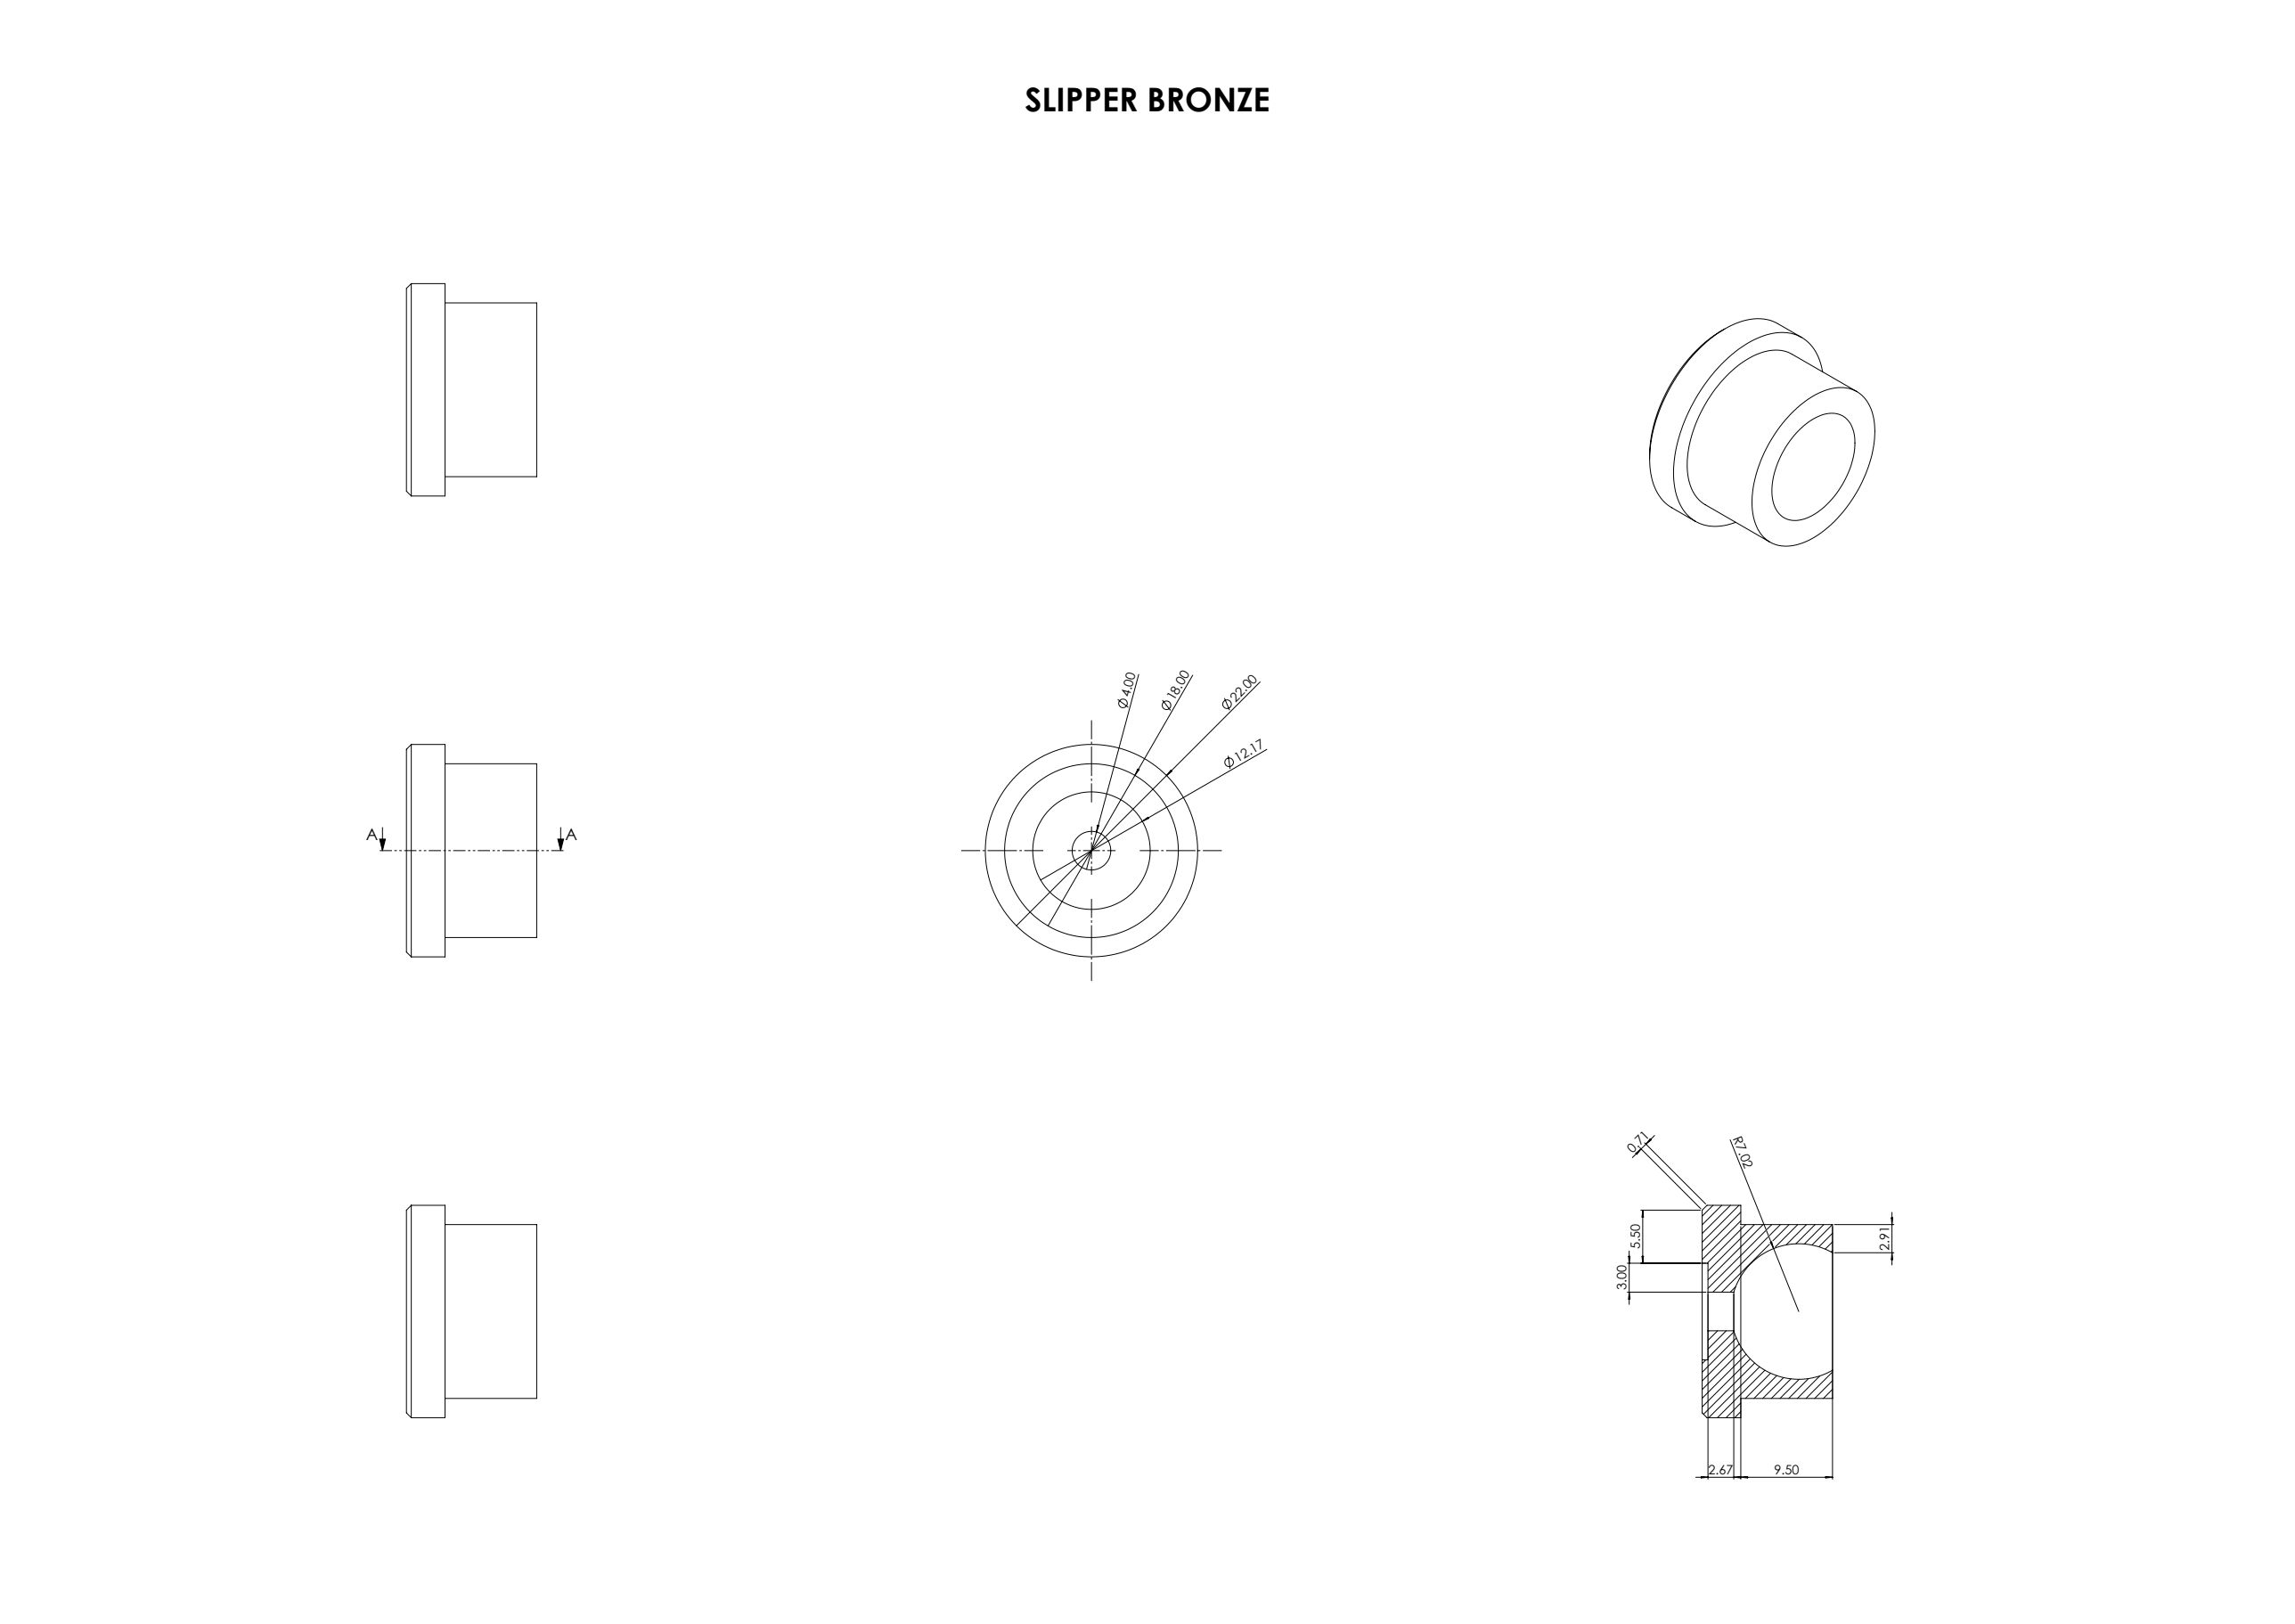
ISO-10303-21;
HEADER;
/* Generated by software containing ST-Developer
 * from STEP Tools, Inc. (www.steptools.com) 
 */

FILE_DESCRIPTION(
/* description */ (''),
/* implementation_level */ '2;1');

FILE_NAME(
/* name */ '06_Slipper_Bronze.step',
/* time_stamp */ '2026-10-26T07:49:00-07:00',
/* author */ (''),
/* organization */ (''),
/* preprocessor_version */ 'ST-DEVELOPER v20.2',
/* originating_system */ 'Autodesk Translation Framework v15.15.0.0',
/* authorisation */ '');

FILE_SCHEMA (('AUTOMOTIVE_DESIGN { 1 0 10303 214 3 1 1 }'));
ENDSEC;

DATA;
#10=MECHANICAL_DESIGN_GEOMETRIC_PRESENTATION_REPRESENTATION('',(#188),#38507);
#146=SPHERICAL_SURFACE('',#16295,7.02);
#158=SHAPE_REPRESENTATION_RELATIONSHIP('SRR','None',#38586,#173);
#173=ADVANCED_BREP_SHAPE_REPRESENTATION('',(#203),#38503);
#188=STYLED_ITEM('',(#38713),#203);
#203=MANIFOLD_SOLID_BREP('Slipper_Body',#15082);
#510=FACE_BOUND('',#3163,.T.);
#511=FACE_BOUND('',#3167,.T.);
#512=FACE_BOUND('',#3170,.T.);
#513=FACE_BOUND('',#3172,.T.);
#514=FACE_BOUND('',#3175,.T.);
#805=PLANE('',#16283);
#806=PLANE('',#16289);
#807=PLANE('',#16293);
#808=PLANE('',#16303);
#1509=CYLINDRICAL_SURFACE('',#16280,5.);
#1510=CYLINDRICAL_SURFACE('',#16287,11.);
#1511=CYLINDRICAL_SURFACE('',#16291,9.);
#1512=CYLINDRICAL_SURFACE('',#16301,2.);
#2181=FACE_OUTER_BOUND('',#3161,.T.);
#2182=FACE_OUTER_BOUND('',#3162,.T.);
#2183=FACE_OUTER_BOUND('',#3164,.T.);
#2184=FACE_OUTER_BOUND('',#3165,.T.);
#2185=FACE_OUTER_BOUND('',#3166,.T.);
#2186=FACE_OUTER_BOUND('',#3168,.T.);
#2187=FACE_OUTER_BOUND('',#3169,.T.);
#2188=FACE_OUTER_BOUND('',#3171,.T.);
#2189=FACE_OUTER_BOUND('',#3173,.T.);
#2190=FACE_OUTER_BOUND('',#3174,.T.);
#3161=EDGE_LOOP('',(#12527,#12528,#12529,#12530));
#3162=EDGE_LOOP('',(#12531));
#3163=EDGE_LOOP('',(#12532));
#3164=EDGE_LOOP('',(#12533,#12534,#12535,#12536));
#3165=EDGE_LOOP('',(#12537,#12538,#12539,#12540));
#3166=EDGE_LOOP('',(#12541));
#3167=EDGE_LOOP('',(#12542));
#3168=EDGE_LOOP('',(#12543,#12544,#12545,#12546));
#3169=EDGE_LOOP('',(#12547));
#3170=EDGE_LOOP('',(#12548));
#3171=EDGE_LOOP('',(#12549,#12550,#12551,#12552,#12553,#12554,#12555));
#3172=EDGE_LOOP('',(#12556));
#3173=EDGE_LOOP('',(#12557,#12558,#12559,#12560,#12561,#12562));
#3174=EDGE_LOOP('',(#12563));
#3175=EDGE_LOOP('',(#12564));
#4136=LINE('',#27087,#5205);
#4137=LINE('',#27095,#5206);
#4138=LINE('',#27099,#5207);
#4139=LINE('',#27106,#5208);
#4140=LINE('',#27123,#5209);
#5205=VECTOR('',#19439,5.);
#5206=VECTOR('',#19450,10.75);
#5207=VECTOR('',#19455,11.);
#5208=VECTOR('',#19464,9.);
#5209=VECTOR('',#19483,2.);
#6128=CIRCLE('',#16281,5.);
#6129=CIRCLE('',#16282,5.);
#6130=CIRCLE('',#16284,10.5);
#6131=CIRCLE('',#16286,11.);
#6132=CIRCLE('',#16288,11.);
#6133=CIRCLE('',#16290,9.);
#6134=CIRCLE('',#16292,9.);
#6135=CIRCLE('',#16294,6.08526088183572);
#6136=CIRCLE('',#16296,2.);
#6137=CIRCLE('',#16297,7.02);
#6138=CIRCLE('',#16298,2.);
#6139=CIRCLE('',#16299,2.);
#6140=CIRCLE('',#16300,7.02);
#6141=CIRCLE('',#16302,2.);
#7132=VERTEX_POINT('',#27084);
#7133=VERTEX_POINT('',#27086);
#7134=VERTEX_POINT('',#27090);
#7135=VERTEX_POINT('',#27093);
#7136=VERTEX_POINT('',#27097);
#7137=VERTEX_POINT('',#27101);
#7138=VERTEX_POINT('',#27104);
#7139=VERTEX_POINT('',#27108);
#7140=VERTEX_POINT('',#27111);
#7141=VERTEX_POINT('',#27112);
#7142=VERTEX_POINT('',#27114);
#7143=VERTEX_POINT('',#27116);
#7144=VERTEX_POINT('',#27119);
#7145=VERTEX_POINT('',#27122);
#9012=EDGE_CURVE('',#7132,#7132,#6128,.T.);
#9013=EDGE_CURVE('',#7132,#7133,#4136,.T.);
#9014=EDGE_CURVE('',#7133,#7133,#6129,.T.);
#9015=EDGE_CURVE('',#7134,#7134,#6130,.T.);
#9016=EDGE_CURVE('',#7135,#7135,#6131,.T.);
#9017=EDGE_CURVE('',#7135,#7134,#4137,.T.);
#9018=EDGE_CURVE('',#7136,#7136,#6132,.T.);
#9019=EDGE_CURVE('',#7136,#7135,#4138,.T.);
#9020=EDGE_CURVE('',#7137,#7137,#6133,.T.);
#9021=EDGE_CURVE('',#7138,#7138,#6134,.T.);
#9022=EDGE_CURVE('',#7138,#7137,#4139,.T.);
#9023=EDGE_CURVE('',#7139,#7139,#6135,.T.);
#9024=EDGE_CURVE('',#7140,#7141,#6136,.T.);
#9025=EDGE_CURVE('',#7140,#7142,#6137,.T.);
#9026=EDGE_CURVE('',#7143,#7140,#6138,.T.);
#9027=EDGE_CURVE('',#7141,#7143,#6139,.T.);
#9028=EDGE_CURVE('',#7144,#7141,#6140,.T.);
#9029=EDGE_CURVE('',#7143,#7145,#4140,.T.);
#9030=EDGE_CURVE('',#7145,#7145,#6141,.T.);
#12527=ORIENTED_EDGE('',*,*,#9012,.T.);
#12528=ORIENTED_EDGE('',*,*,#9013,.T.);
#12529=ORIENTED_EDGE('',*,*,#9014,.F.);
#12530=ORIENTED_EDGE('',*,*,#9013,.F.);
#12531=ORIENTED_EDGE('',*,*,#9015,.F.);
#12532=ORIENTED_EDGE('',*,*,#9014,.T.);
#12533=ORIENTED_EDGE('',*,*,#9016,.F.);
#12534=ORIENTED_EDGE('',*,*,#9017,.T.);
#12535=ORIENTED_EDGE('',*,*,#9015,.T.);
#12536=ORIENTED_EDGE('',*,*,#9017,.F.);
#12537=ORIENTED_EDGE('',*,*,#9018,.F.);
#12538=ORIENTED_EDGE('',*,*,#9019,.T.);
#12539=ORIENTED_EDGE('',*,*,#9016,.T.);
#12540=ORIENTED_EDGE('',*,*,#9019,.F.);
#12541=ORIENTED_EDGE('',*,*,#9018,.T.);
#12542=ORIENTED_EDGE('',*,*,#9020,.F.);
#12543=ORIENTED_EDGE('',*,*,#9021,.F.);
#12544=ORIENTED_EDGE('',*,*,#9022,.T.);
#12545=ORIENTED_EDGE('',*,*,#9020,.T.);
#12546=ORIENTED_EDGE('',*,*,#9022,.F.);
#12547=ORIENTED_EDGE('',*,*,#9021,.T.);
#12548=ORIENTED_EDGE('',*,*,#9023,.F.);
#12549=ORIENTED_EDGE('',*,*,#9024,.F.);
#12550=ORIENTED_EDGE('',*,*,#9025,.T.);
#12551=ORIENTED_EDGE('',*,*,#9025,.F.);
#12552=ORIENTED_EDGE('',*,*,#9026,.F.);
#12553=ORIENTED_EDGE('',*,*,#9027,.F.);
#12554=ORIENTED_EDGE('',*,*,#9028,.F.);
#12555=ORIENTED_EDGE('',*,*,#9028,.T.);
#12556=ORIENTED_EDGE('',*,*,#9023,.T.);
#12557=ORIENTED_EDGE('',*,*,#9024,.T.);
#12558=ORIENTED_EDGE('',*,*,#9027,.T.);
#12559=ORIENTED_EDGE('',*,*,#9029,.T.);
#12560=ORIENTED_EDGE('',*,*,#9030,.F.);
#12561=ORIENTED_EDGE('',*,*,#9029,.F.);
#12562=ORIENTED_EDGE('',*,*,#9026,.T.);
#12563=ORIENTED_EDGE('',*,*,#9012,.F.);
#12564=ORIENTED_EDGE('',*,*,#9030,.T.);
#14178=CONICAL_SURFACE('',#16285,10.75,0.785398163397449);
#14748=ADVANCED_FACE('',(#2181),#1509,.F.);
#14749=ADVANCED_FACE('',(#2182,#510),#805,.T.);
#14750=ADVANCED_FACE('',(#2183),#14178,.T.);
#14751=ADVANCED_FACE('',(#2184),#1510,.T.);
#14752=ADVANCED_FACE('',(#2185,#511),#806,.T.);
#14753=ADVANCED_FACE('',(#2186),#1511,.T.);
#14754=ADVANCED_FACE('',(#2187,#512),#807,.T.);
#14755=ADVANCED_FACE('',(#2188,#513),#146,.F.);
#14756=ADVANCED_FACE('',(#2189),#1512,.F.);
#14757=ADVANCED_FACE('',(#2190,#514),#808,.T.);
#15082=CLOSED_SHELL('',(#14748,#14749,#14750,#14751,#14752,#14753,#14754,
#14755,#14756,#14757));
#16279=AXIS2_PLACEMENT_3D('',#27082,#19433,#19434);
#16280=AXIS2_PLACEMENT_3D('',#27083,#19435,#19436);
#16281=AXIS2_PLACEMENT_3D('',#27085,#19437,#19438);
#16282=AXIS2_PLACEMENT_3D('',#27088,#19440,#19441);
#16283=AXIS2_PLACEMENT_3D('',#27089,#19442,#19443);
#16284=AXIS2_PLACEMENT_3D('',#27091,#19444,#19445);
#16285=AXIS2_PLACEMENT_3D('',#27092,#19446,#19447);
#16286=AXIS2_PLACEMENT_3D('',#27094,#19448,#19449);
#16287=AXIS2_PLACEMENT_3D('',#27096,#19451,#19452);
#16288=AXIS2_PLACEMENT_3D('',#27098,#19453,#19454);
#16289=AXIS2_PLACEMENT_3D('',#27100,#19456,#19457);
#16290=AXIS2_PLACEMENT_3D('',#27102,#19458,#19459);
#16291=AXIS2_PLACEMENT_3D('',#27103,#19460,#19461);
#16292=AXIS2_PLACEMENT_3D('',#27105,#19462,#19463);
#16293=AXIS2_PLACEMENT_3D('',#27107,#19465,#19466);
#16294=AXIS2_PLACEMENT_3D('',#27109,#19467,#19468);
#16295=AXIS2_PLACEMENT_3D('',#27110,#19469,#19470);
#16296=AXIS2_PLACEMENT_3D('',#27113,#19471,#19472);
#16297=AXIS2_PLACEMENT_3D('',#27115,#19473,#19474);
#16298=AXIS2_PLACEMENT_3D('',#27117,#19475,#19476);
#16299=AXIS2_PLACEMENT_3D('',#27118,#19477,#19478);
#16300=AXIS2_PLACEMENT_3D('',#27120,#19479,#19480);
#16301=AXIS2_PLACEMENT_3D('',#27121,#19481,#19482);
#16302=AXIS2_PLACEMENT_3D('',#27124,#19484,#19485);
#16303=AXIS2_PLACEMENT_3D('',#27125,#19486,#19487);
#19433=DIRECTION('axis',(0.,0.,1.));
#19434=DIRECTION('refdir',(1.,0.,0.));
#19435=DIRECTION('center_axis',(1.,0.,0.));
#19436=DIRECTION('ref_axis',(0.,1.,0.));
#19437=DIRECTION('center_axis',(1.,0.,0.));
#19438=DIRECTION('ref_axis',(0.,0.,-1.));
#19439=DIRECTION('',(-1.,0.,0.));
#19440=DIRECTION('center_axis',(1.,0.,0.));
#19441=DIRECTION('ref_axis',(0.,0.,-1.));
#19442=DIRECTION('center_axis',(-1.,0.,0.));
#19443=DIRECTION('ref_axis',(0.,0.,1.));
#19444=DIRECTION('center_axis',(1.,0.,0.));
#19445=DIRECTION('ref_axis',(0.,0.,-1.));
#19446=DIRECTION('center_axis',(1.,0.,0.));
#19447=DIRECTION('ref_axis',(0.,1.,0.));
#19448=DIRECTION('center_axis',(1.,0.,0.));
#19449=DIRECTION('ref_axis',(0.,0.,-1.));
#19450=DIRECTION('',(-0.707106781186547,0.707106781186548,8.65956056235494E-17));
#19451=DIRECTION('center_axis',(1.,0.,0.));
#19452=DIRECTION('ref_axis',(0.,1.,0.));
#19453=DIRECTION('center_axis',(1.,0.,0.));
#19454=DIRECTION('ref_axis',(0.,0.,-1.));
#19455=DIRECTION('',(-1.,0.,0.));
#19456=DIRECTION('center_axis',(1.,0.,0.));
#19457=DIRECTION('ref_axis',(0.,0.,-1.));
#19458=DIRECTION('center_axis',(1.,0.,0.));
#19459=DIRECTION('ref_axis',(0.,0.,-1.));
#19460=DIRECTION('center_axis',(1.,0.,0.));
#19461=DIRECTION('ref_axis',(0.,1.,0.));
#19462=DIRECTION('center_axis',(1.,0.,0.));
#19463=DIRECTION('ref_axis',(0.,0.,-1.));
#19464=DIRECTION('',(-1.,0.,0.));
#19465=DIRECTION('center_axis',(1.,0.,0.));
#19466=DIRECTION('ref_axis',(0.,0.,-1.));
#19467=DIRECTION('center_axis',(1.,0.,0.));
#19468=DIRECTION('ref_axis',(0.,0.,-1.));
#19469=DIRECTION('center_axis',(0.,0.,1.));
#19470=DIRECTION('ref_axis',(1.,0.,0.));
#19471=DIRECTION('center_axis',(1.,0.,0.));
#19472=DIRECTION('ref_axis',(0.,0.,-1.));
#19473=DIRECTION('center_axis',(1.22464679914735E-16,-1.,0.));
#19474=DIRECTION('ref_axis',(-1.,-1.22464679914735E-16,0.));
#19475=DIRECTION('center_axis',(1.,0.,0.));
#19476=DIRECTION('ref_axis',(0.,0.,-1.));
#19477=DIRECTION('center_axis',(1.,0.,0.));
#19478=DIRECTION('ref_axis',(0.,0.,-1.));
#19479=DIRECTION('center_axis',(1.22464679914735E-16,-1.,0.));
#19480=DIRECTION('ref_axis',(-1.,-1.22464679914735E-16,0.));
#19481=DIRECTION('center_axis',(1.,0.,0.));
#19482=DIRECTION('ref_axis',(0.,1.,0.));
#19483=DIRECTION('',(-1.,0.,0.));
#19484=DIRECTION('center_axis',(1.,0.,0.));
#19485=DIRECTION('ref_axis',(0.,0.,-1.));
#19486=DIRECTION('center_axis',(-1.,0.,0.));
#19487=DIRECTION('ref_axis',(0.,0.,1.));
#27082=CARTESIAN_POINT('',(0.,0.,0.));
#27083=CARTESIAN_POINT('Origin',(0.3,0.,0.));
#27084=CARTESIAN_POINT('',(0.6,-5.,-6.12323399573677E-16));
#27085=CARTESIAN_POINT('Origin',(0.6,0.,0.));
#27086=CARTESIAN_POINT('',(0.,-5.,-6.12323399573677E-16));
#27087=CARTESIAN_POINT('',(0.3,-5.,-6.12323399573677E-16));
#27088=CARTESIAN_POINT('Origin',(0.,0.,0.));
#27089=CARTESIAN_POINT('Origin',(0.,10.5,0.));
#27090=CARTESIAN_POINT('',(-7.97972798949331E-16,-10.5,-1.28587913910472E-15));
#27091=CARTESIAN_POINT('Origin',(0.,0.,0.));
#27092=CARTESIAN_POINT('Origin',(0.25,0.,0.));
#27093=CARTESIAN_POINT('',(0.5,-11.,-1.34711147906209E-15));
#27094=CARTESIAN_POINT('Origin',(0.5,0.,0.));
#27095=CARTESIAN_POINT('',(0.25,-10.75,-1.3164953090834E-15));
#27096=CARTESIAN_POINT('Origin',(2.25,0.,0.));
#27097=CARTESIAN_POINT('',(4.,-11.,-1.34711147906209E-15));
#27098=CARTESIAN_POINT('Origin',(4.,0.,0.));
#27099=CARTESIAN_POINT('',(2.25,-11.,-1.34711147906209E-15));
#27100=CARTESIAN_POINT('Origin',(4.,9.,0.));
#27101=CARTESIAN_POINT('',(4.,-9.,-1.10218211923262E-15));
#27102=CARTESIAN_POINT('Origin',(4.,0.,0.));
#27103=CARTESIAN_POINT('Origin',(8.75,0.,0.));
#27104=CARTESIAN_POINT('',(13.5,-9.,-1.10218211923262E-15));
#27105=CARTESIAN_POINT('Origin',(13.5,0.,0.));
#27106=CARTESIAN_POINT('',(8.75,-9.,-1.10218211923262E-15));
#27107=CARTESIAN_POINT('Origin',(13.5,6.08526088183572,0.));
#27108=CARTESIAN_POINT('',(13.5,6.08526088183572,0.));
#27109=CARTESIAN_POINT('Origin',(13.5,0.,0.));
#27110=CARTESIAN_POINT('Origin',(10.,-1.11022302462516E-15,0.));
#27111=CARTESIAN_POINT('',(3.27092874164644,-1.93429658240287E-15,-2.));
#27112=CARTESIAN_POINT('',(3.27092874164644,-1.93429658240287E-15,2.));
#27113=CARTESIAN_POINT('Origin',(3.27092874164644,0.,0.));
#27114=CARTESIAN_POINT('',(10.,-1.11022302462516E-15,-7.02));
#27115=CARTESIAN_POINT('Origin',(10.,-1.11022302462516E-15,0.));
#27116=CARTESIAN_POINT('',(3.27092874164644,-2.,-2.44929359829471E-16));
#27117=CARTESIAN_POINT('Origin',(3.27092874164644,0.,0.));
#27118=CARTESIAN_POINT('Origin',(3.27092874164644,0.,0.));
#27119=CARTESIAN_POINT('',(10.,-1.11022302462516E-15,7.02));
#27120=CARTESIAN_POINT('Origin',(10.,-1.11022302462516E-15,0.));
#27121=CARTESIAN_POINT('Origin',(1.93546437082322,0.,0.));
#27122=CARTESIAN_POINT('',(0.6,-2.,-2.44929359829471E-16));
#27123=CARTESIAN_POINT('',(1.93546437082322,-2.,-2.44929359829471E-16));
#27124=CARTESIAN_POINT('Origin',(0.6,0.,0.));
#27125=CARTESIAN_POINT('Origin',(0.6,5.,0.));
#38486=UNCERTAINTY_MEASURE_WITH_UNIT(LENGTH_MEASURE(0.01),#38508,
'DISTANCE_ACCURACY_VALUE',
'Maximum model space distance between geometric entities at asserted c
onnectivities');
#38490=UNCERTAINTY_MEASURE_WITH_UNIT(LENGTH_MEASURE(0.01),#38508,
'DISTANCE_ACCURACY_VALUE',
'Maximum model space distance between geometric entities at asserted c
onnectivities');
#38503=(
GEOMETRIC_REPRESENTATION_CONTEXT(3)
GLOBAL_UNCERTAINTY_ASSIGNED_CONTEXT((#38486))
GLOBAL_UNIT_ASSIGNED_CONTEXT((#38508,#38510,#38511))
REPRESENTATION_CONTEXT('','3D')
);
#38507=(
GEOMETRIC_REPRESENTATION_CONTEXT(3)
GLOBAL_UNCERTAINTY_ASSIGNED_CONTEXT((#38490))
GLOBAL_UNIT_ASSIGNED_CONTEXT((#38508,#38510,#38511))
REPRESENTATION_CONTEXT('','3D')
);
#38508=(
LENGTH_UNIT()
NAMED_UNIT(*)
SI_UNIT(.MILLI.,.METRE.)
);
#38510=(
NAMED_UNIT(*)
PLANE_ANGLE_UNIT()
SI_UNIT($,.RADIAN.)
);
#38511=(
NAMED_UNIT(*)
SI_UNIT($,.STERADIAN.)
SOLID_ANGLE_UNIT()
);
#38524=SHAPE_DEFINITION_REPRESENTATION(#38540,#38586);
#38540=PRODUCT_DEFINITION_SHAPE('',$,#38603);
#38586=SHAPE_REPRESENTATION('',(#16279),#38503);
#38590=PRODUCT_DEFINITION_CONTEXT('part definition',#38640,'design');
#38603=PRODUCT_DEFINITION('2026-10-26-01-10-49-065','06_Slipper_Bronze',
#38619,#38590);
#38619=PRODUCT_DEFINITION_FORMATION('',$,#38654);
#38640=APPLICATION_CONTEXT(
'Core Data for Automotive Mechanical Design Process');
#38641=PRODUCT_CONTEXT('part definition',#38640,'mechanical');
#38654=PRODUCT('2026-10-26-01-10-49-065','06_Slipper_Bronze',$,(#38641));
#38707=COLOUR_RGB('Sky Blue',0.24,0.69,0.87);
#38708=FILL_AREA_STYLE_COLOUR('',#38707);
#38709=FILL_AREA_STYLE('',(#38708));
#38710=SURFACE_STYLE_FILL_AREA(#38709);
#38711=SURFACE_SIDE_STYLE('',(#38710));
#38712=SURFACE_STYLE_USAGE(.BOTH.,#38711);
#38713=PRESENTATION_STYLE_ASSIGNMENT((#38712));
ENDSEC;
END-ISO-10303-21;
